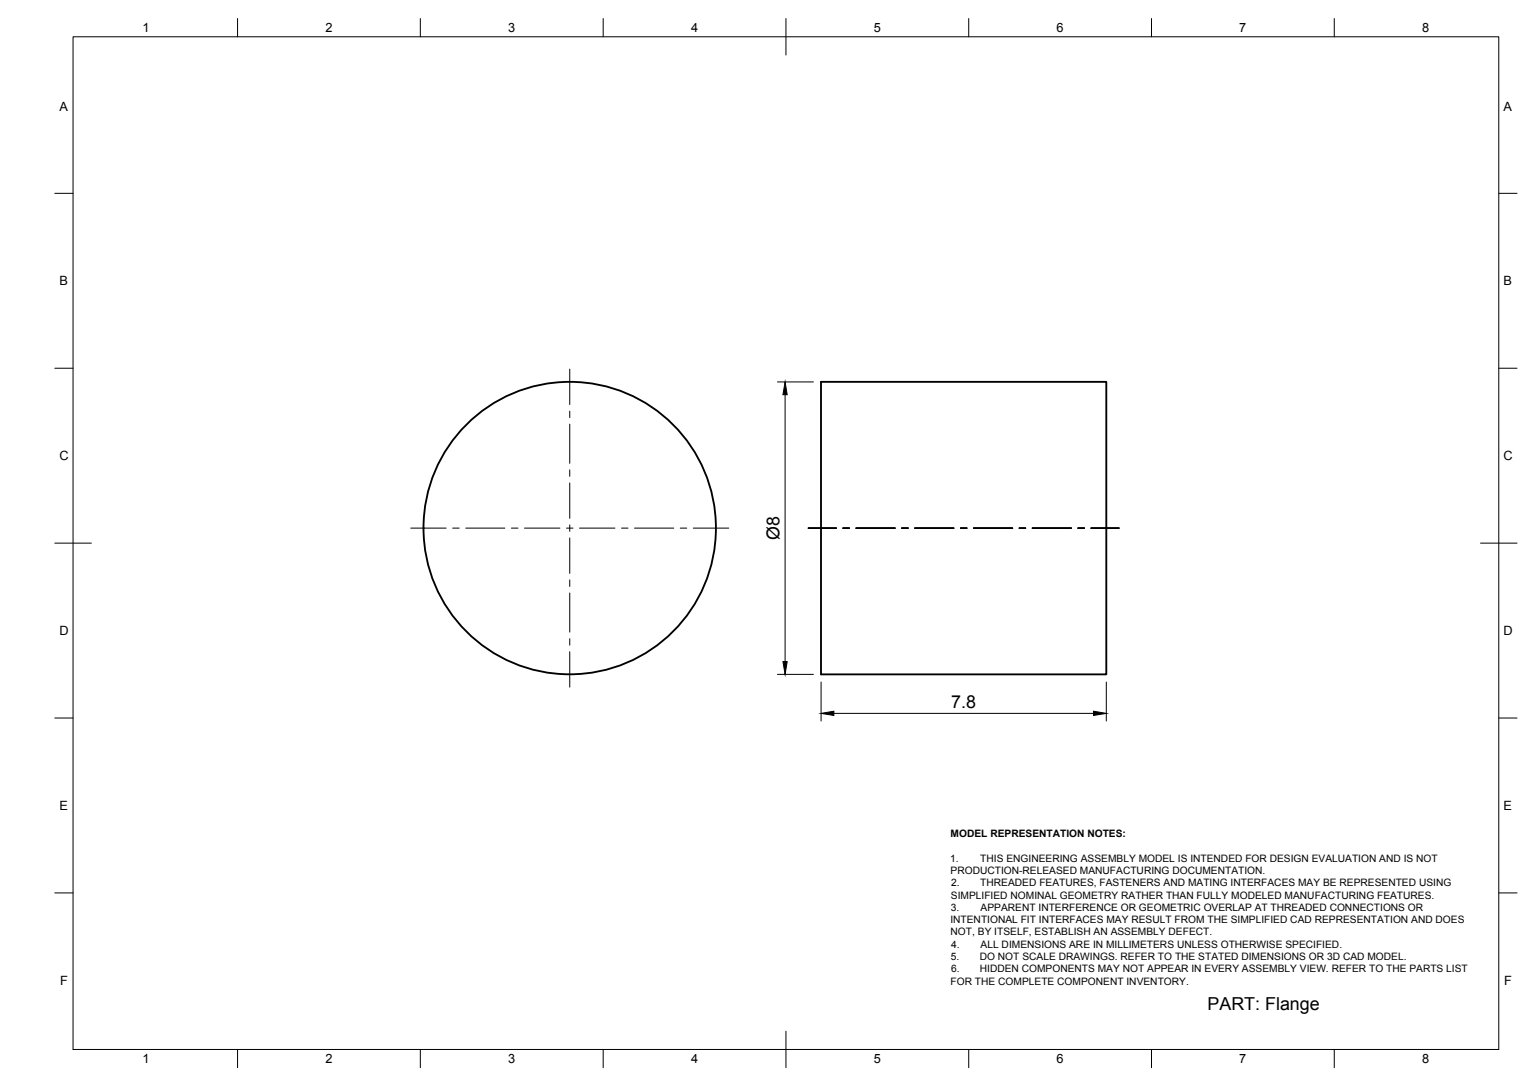
ISO-10303-21;
HEADER;
/* Generated by software containing ST-Developer
 * from STEP Tools, Inc. (www.steptools.com) 
 */

FILE_DESCRIPTION(
/* description */ (''),
/* implementation_level */ '2;1');

FILE_NAME(
/* name */ 'Flange.step',
/* time_stamp */ '2026-10-05T01:33:24-07:00',
/* author */ (''),
/* organization */ (''),
/* preprocessor_version */ 'ST-DEVELOPER v20.2',
/* originating_system */ 'Autodesk Translation Framework v15.15.0.0',
/* authorisation */ '');

FILE_SCHEMA (('AUTOMOTIVE_DESIGN { 1 0 10303 214 3 1 1 }'));
ENDSEC;

DATA;
#10=MECHANICAL_DESIGN_GEOMETRIC_PRESENTATION_REPRESENTATION('',(#86),#1128);
#66=SHAPE_REPRESENTATION_RELATIONSHIP('SRR','None',#1170,#76);
#76=ADVANCED_BREP_SHAPE_REPRESENTATION('',(#96),#1122);
#86=STYLED_ITEM('',(#1227),#96);
#96=MANIFOLD_SOLID_BREP('Body1',#525);
#109=LINE('',#1025,#126);
#126=VECTOR('',#840,4.);
#140=CYLINDRICAL_SURFACE('',#687,4.);
#164=FACE_OUTER_BOUND('',#205,.T.);
#165=FACE_OUTER_BOUND('',#206,.T.);
#166=FACE_OUTER_BOUND('',#207,.T.);
#205=EDGE_LOOP('',(#400));
#206=EDGE_LOOP('',(#401));
#207=EDGE_LOOP('',(#402,#403,#404,#405));
#245=CIRCLE('',#684,4.);
#246=CIRCLE('',#686,4.);
#279=VERTEX_POINT('',#1019);
#280=VERTEX_POINT('',#1022);
#322=EDGE_CURVE('',#279,#279,#245,.T.);
#323=EDGE_CURVE('',#280,#280,#246,.T.);
#324=EDGE_CURVE('',#279,#280,#109,.T.);
#400=ORIENTED_EDGE('',*,*,#322,.T.);
#401=ORIENTED_EDGE('',*,*,#323,.F.);
#402=ORIENTED_EDGE('',*,*,#322,.F.);
#403=ORIENTED_EDGE('',*,*,#324,.T.);
#404=ORIENTED_EDGE('',*,*,#323,.T.);
#405=ORIENTED_EDGE('',*,*,#324,.F.);
#468=PLANE('',#683);
#469=PLANE('',#685);
#498=ADVANCED_FACE('',(#164),#468,.T.);
#499=ADVANCED_FACE('',(#165),#469,.T.);
#500=ADVANCED_FACE('',(#166),#140,.T.);
#525=CLOSED_SHELL('',(#498,#499,#500));
#682=AXIS2_PLACEMENT_3D('',#1017,#828,#829);
#683=AXIS2_PLACEMENT_3D('',#1018,#830,#831);
#684=AXIS2_PLACEMENT_3D('',#1020,#832,#833);
#685=AXIS2_PLACEMENT_3D('',#1021,#834,#835);
#686=AXIS2_PLACEMENT_3D('',#1023,#836,#837);
#687=AXIS2_PLACEMENT_3D('',#1024,#838,#839);
#828=DIRECTION('axis',(0.,0.,1.));
#829=DIRECTION('refdir',(1.,0.,0.));
#830=DIRECTION('center_axis',(1.,0.,0.));
#831=DIRECTION('ref_axis',(0.,0.,-1.));
#832=DIRECTION('center_axis',(1.,0.,0.));
#833=DIRECTION('ref_axis',(0.,0.,-1.));
#834=DIRECTION('center_axis',(-1.,0.,0.));
#835=DIRECTION('ref_axis',(0.,0.,1.));
#836=DIRECTION('center_axis',(1.,0.,0.));
#837=DIRECTION('ref_axis',(0.,0.,-1.));
#838=DIRECTION('center_axis',(1.,0.,0.));
#839=DIRECTION('ref_axis',(0.,0.,-1.));
#840=DIRECTION('',(-1.,0.,0.));
#1017=CARTESIAN_POINT('',(0.,0.,0.));
#1018=CARTESIAN_POINT('Origin',(31.0379185953459,0.,0.));
#1019=CARTESIAN_POINT('',(31.0379185953459,-4.89858719658941E-16,4.));
#1020=CARTESIAN_POINT('Origin',(31.0379185953459,0.,0.));
#1021=CARTESIAN_POINT('Origin',(23.2354431734887,0.,-4.));
#1022=CARTESIAN_POINT('',(23.2354431734887,-4.89858719658941E-16,4.));
#1023=CARTESIAN_POINT('Origin',(23.2354431734887,0.,0.));
#1024=CARTESIAN_POINT('Origin',(27.1366808844173,0.,0.));
#1025=CARTESIAN_POINT('',(27.1366808844173,-4.89858719658941E-16,4.));
#1110=UNCERTAINTY_MEASURE_WITH_UNIT(LENGTH_MEASURE(0.01),#1129,
'DISTANCE_ACCURACY_VALUE',
'Maximum model space distance between geometric entities at asserted c
onnectivities');
#1116=UNCERTAINTY_MEASURE_WITH_UNIT(LENGTH_MEASURE(0.01),#1129,
'DISTANCE_ACCURACY_VALUE',
'Maximum model space distance between geometric entities at asserted c
onnectivities');
#1122=(
GEOMETRIC_REPRESENTATION_CONTEXT(3)
GLOBAL_UNCERTAINTY_ASSIGNED_CONTEXT((#1110))
GLOBAL_UNIT_ASSIGNED_CONTEXT((#1129,#1131,#1132))
REPRESENTATION_CONTEXT('','3D')
);
#1128=(
GEOMETRIC_REPRESENTATION_CONTEXT(3)
GLOBAL_UNCERTAINTY_ASSIGNED_CONTEXT((#1116))
GLOBAL_UNIT_ASSIGNED_CONTEXT((#1129,#1131,#1132))
REPRESENTATION_CONTEXT('','3D')
);
#1129=(
LENGTH_UNIT()
NAMED_UNIT(*)
SI_UNIT(.MILLI.,.METRE.)
);
#1131=(
NAMED_UNIT(*)
PLANE_ANGLE_UNIT()
SI_UNIT($,.RADIAN.)
);
#1132=(
NAMED_UNIT(*)
SI_UNIT($,.STERADIAN.)
SOLID_ANGLE_UNIT()
);
#1138=SHAPE_DEFINITION_REPRESENTATION(#1149,#1170);
#1149=PRODUCT_DEFINITION_SHAPE('',$,#1182);
#1170=SHAPE_REPRESENTATION('',(#682),#1122);
#1176=PRODUCT_DEFINITION_CONTEXT('part definition',#1211,'design');
#1182=PRODUCT_DEFINITION('Flange','Flange',#1193,#1176);
#1193=PRODUCT_DEFINITION_FORMATION('',$,#1218);
#1211=APPLICATION_CONTEXT(
'Core Data for Automotive Mechanical Design Process');
#1212=PRODUCT_CONTEXT('part definition',#1211,'mechanical');
#1218=PRODUCT('Flange','Flange',$,(#1212));
#1227=PRESENTATION_STYLE_ASSIGNMENT((#1231));
#1231=SURFACE_STYLE_USAGE(.BOTH.,#1235);
#1235=SURFACE_SIDE_STYLE('',(#1239));
#1239=SURFACE_STYLE_FILL_AREA(#1243);
#1243=FILL_AREA_STYLE('Opaque(77,77,77)',(#1247));
#1247=FILL_AREA_STYLE_COLOUR('Opaque(77,77,77)',#1251);
#1251=COLOUR_RGB('Opaque(77,77,77)', 0.72549020, 0.75294118, 0.79215686);
ENDSEC;
END-ISO-10303-21;
